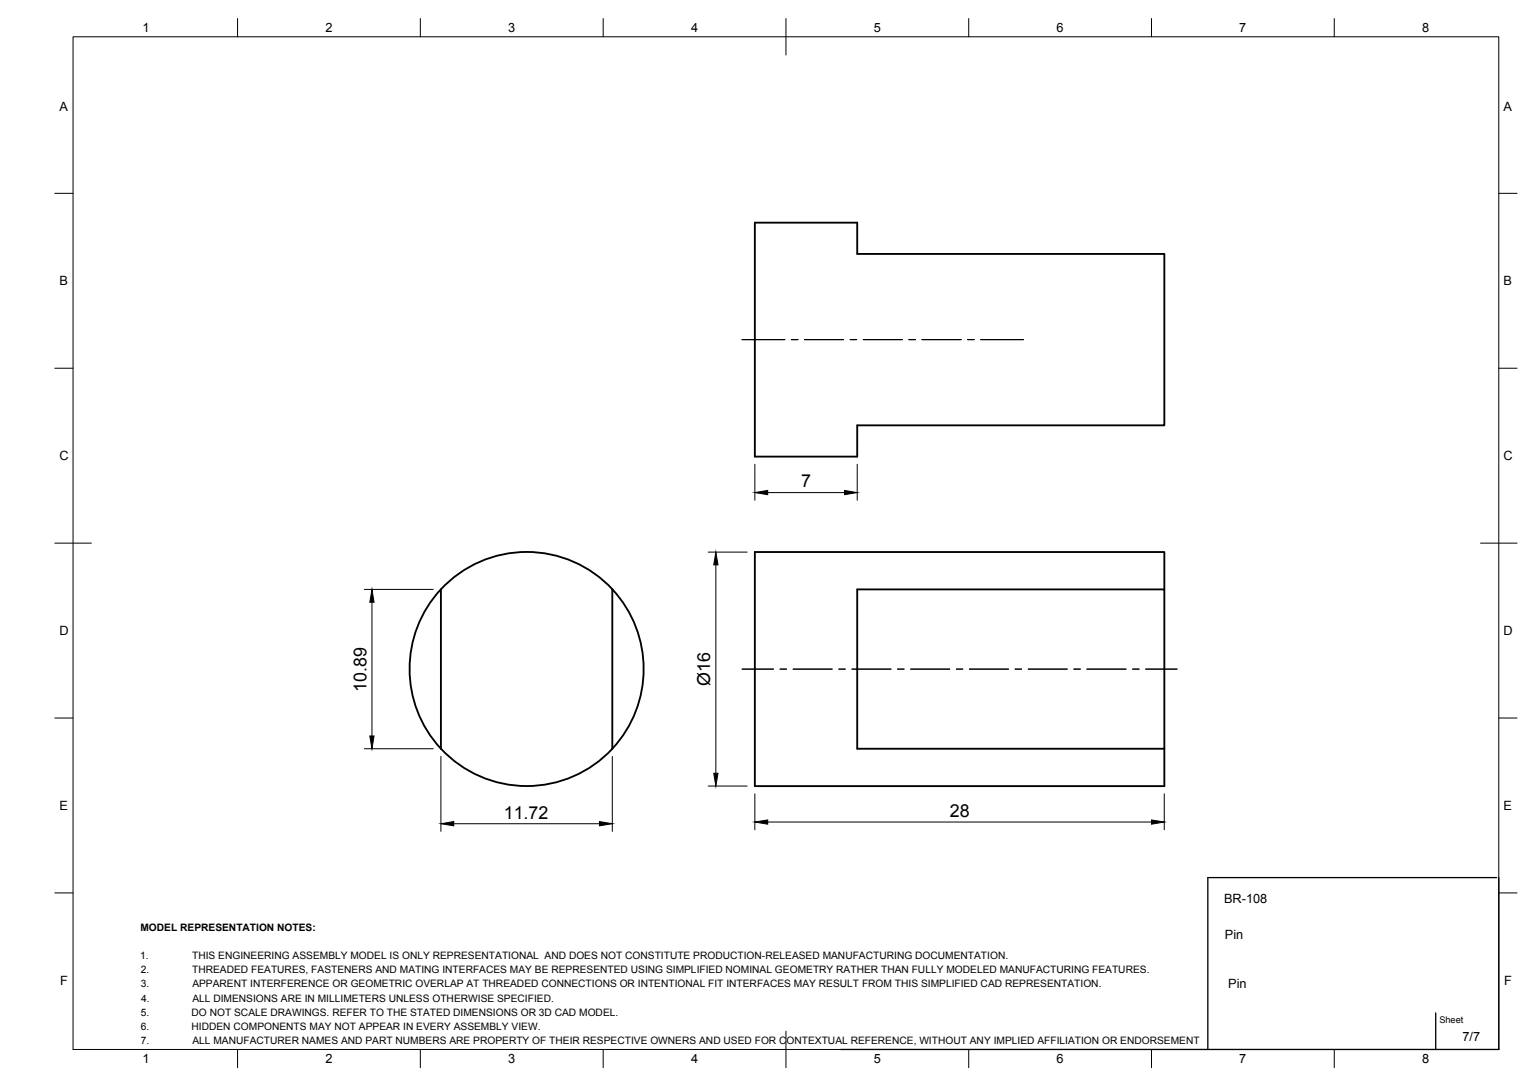
ISO-10303-21;
HEADER;
/* Generated by software containing ST-Developer
 * from STEP Tools, Inc. (www.steptools.com) 
 */

FILE_DESCRIPTION(
/* description */ (''),
/* implementation_level */ '2;1');

FILE_NAME(
/* name */ 'Pin.step',
/* time_stamp */ '2026-11-14T03:52:36-08:00',
/* author */ (''),
/* organization */ (''),
/* preprocessor_version */ 'ST-DEVELOPER v20.2',
/* originating_system */ 'Autodesk Translation Framework v15.17.0.0',
/* authorisation */ '');

FILE_SCHEMA (('AUTOMOTIVE_DESIGN { 1 0 10303 214 3 1 1 }'));
ENDSEC;

DATA;
#10=MECHANICAL_DESIGN_GEOMETRIC_PRESENTATION_REPRESENTATION('',(#197),#19443);
#181=SHAPE_REPRESENTATION_RELATIONSHIP('SRR','None',#19481,#189);
#189=ADVANCED_BREP_SHAPE_REPRESENTATION('',(#205),#19441);
#197=STYLED_ITEM('',(#19525),#205);
#205=MANIFOLD_SOLID_BREP('Body1',#2024);
#259=PLANE('',#2233);
#260=PLANE('',#2235);
#261=PLANE('',#2237);
#262=PLANE('',#2239);
#263=PLANE('',#2244);
#264=PLANE('',#2245);
#353=FACE_OUTER_BOUND('',#460,.T.);
#354=FACE_OUTER_BOUND('',#461,.T.);
#355=FACE_OUTER_BOUND('',#462,.T.);
#356=FACE_OUTER_BOUND('',#463,.T.);
#357=FACE_OUTER_BOUND('',#464,.T.);
#358=FACE_OUTER_BOUND('',#465,.T.);
#359=FACE_OUTER_BOUND('',#466,.T.);
#460=EDGE_LOOP('',(#1813,#1814));
#461=EDGE_LOOP('',(#1815,#1816));
#462=EDGE_LOOP('',(#1817));
#463=EDGE_LOOP('',(#1818,#1819,#1820,#1821));
#464=EDGE_LOOP('',(#1822,#1823,#1824,#1825,#1826,#1827,#1828,#1829,#1830,
#1831,#1832,#1833));
#465=EDGE_LOOP('',(#1834,#1835,#1836,#1837));
#466=EDGE_LOOP('',(#1838,#1839,#1840,#1841,#1842));
#577=LINE('',#19342,#704);
#578=LINE('',#19347,#705);
#579=LINE('',#19354,#706);
#580=LINE('',#19356,#707);
#581=LINE('',#19357,#708);
#582=LINE('',#19363,#709);
#583=LINE('',#19365,#710);
#584=LINE('',#19367,#711);
#585=LINE('',#19369,#712);
#704=VECTOR('',#2603,10.);
#705=VECTOR('',#2608,10.);
#706=VECTOR('',#2617,10.);
#707=VECTOR('',#2618,10.);
#708=VECTOR('',#2619,10.);
#709=VECTOR('',#2626,10.);
#710=VECTOR('',#2627,10.);
#711=VECTOR('',#2630,8.);
#712=VECTOR('',#2633,10.);
#768=CIRCLE('',#2234,8.);
#769=CIRCLE('',#2236,8.);
#770=CIRCLE('',#2238,8.);
#771=CIRCLE('',#2241,8.);
#772=CIRCLE('',#2242,8.);
#773=CIRCLE('',#2243,8.);
#970=VERTEX_POINT('',#19340);
#971=VERTEX_POINT('',#19341);
#972=VERTEX_POINT('',#19345);
#973=VERTEX_POINT('',#19346);
#974=VERTEX_POINT('',#19350);
#975=VERTEX_POINT('',#19353);
#976=VERTEX_POINT('',#19355);
#977=VERTEX_POINT('',#19359);
#978=VERTEX_POINT('',#19361);
#979=VERTEX_POINT('',#19364);
#1255=EDGE_CURVE('',#970,#971,#577,.T.);
#1256=EDGE_CURVE('',#971,#970,#768,.T.);
#1257=EDGE_CURVE('',#972,#973,#578,.T.);
#1258=EDGE_CURVE('',#973,#972,#769,.T.);
#1259=EDGE_CURVE('',#974,#974,#770,.T.);
#1260=EDGE_CURVE('',#970,#975,#579,.T.);
#1261=EDGE_CURVE('',#976,#975,#580,.T.);
#1262=EDGE_CURVE('',#971,#976,#581,.T.);
#1263=EDGE_CURVE('',#975,#977,#771,.T.);
#1264=EDGE_CURVE('',#978,#976,#772,.T.);
#1265=EDGE_CURVE('',#972,#978,#582,.T.);
#1266=EDGE_CURVE('',#973,#979,#583,.T.);
#1267=EDGE_CURVE('',#977,#979,#773,.T.);
#1268=EDGE_CURVE('',#977,#974,#584,.T.);
#1269=EDGE_CURVE('',#979,#978,#585,.T.);
#1813=ORIENTED_EDGE('',*,*,#1255,.T.);
#1814=ORIENTED_EDGE('',*,*,#1256,.T.);
#1815=ORIENTED_EDGE('',*,*,#1257,.T.);
#1816=ORIENTED_EDGE('',*,*,#1258,.T.);
#1817=ORIENTED_EDGE('',*,*,#1259,.T.);
#1818=ORIENTED_EDGE('',*,*,#1255,.F.);
#1819=ORIENTED_EDGE('',*,*,#1260,.T.);
#1820=ORIENTED_EDGE('',*,*,#1261,.F.);
#1821=ORIENTED_EDGE('',*,*,#1262,.F.);
#1822=ORIENTED_EDGE('',*,*,#1263,.F.);
#1823=ORIENTED_EDGE('',*,*,#1260,.F.);
#1824=ORIENTED_EDGE('',*,*,#1256,.F.);
#1825=ORIENTED_EDGE('',*,*,#1262,.T.);
#1826=ORIENTED_EDGE('',*,*,#1264,.F.);
#1827=ORIENTED_EDGE('',*,*,#1265,.F.);
#1828=ORIENTED_EDGE('',*,*,#1258,.F.);
#1829=ORIENTED_EDGE('',*,*,#1266,.T.);
#1830=ORIENTED_EDGE('',*,*,#1267,.F.);
#1831=ORIENTED_EDGE('',*,*,#1268,.T.);
#1832=ORIENTED_EDGE('',*,*,#1259,.F.);
#1833=ORIENTED_EDGE('',*,*,#1268,.F.);
#1834=ORIENTED_EDGE('',*,*,#1257,.F.);
#1835=ORIENTED_EDGE('',*,*,#1265,.T.);
#1836=ORIENTED_EDGE('',*,*,#1269,.F.);
#1837=ORIENTED_EDGE('',*,*,#1266,.F.);
#1838=ORIENTED_EDGE('',*,*,#1263,.T.);
#1839=ORIENTED_EDGE('',*,*,#1267,.T.);
#1840=ORIENTED_EDGE('',*,*,#1269,.T.);
#1841=ORIENTED_EDGE('',*,*,#1264,.T.);
#1842=ORIENTED_EDGE('',*,*,#1261,.T.);
#1920=CYLINDRICAL_SURFACE('',#2240,8.);
#2002=ADVANCED_FACE('',(#353),#259,.T.);
#2003=ADVANCED_FACE('',(#354),#260,.T.);
#2004=ADVANCED_FACE('',(#355),#261,.F.);
#2005=ADVANCED_FACE('',(#356),#262,.T.);
#2006=ADVANCED_FACE('',(#357),#1920,.T.);
#2007=ADVANCED_FACE('',(#358),#263,.T.);
#2008=ADVANCED_FACE('',(#359),#264,.T.);
#2024=CLOSED_SHELL('',(#2002,#2003,#2004,#2005,#2006,#2007,#2008));
#2232=AXIS2_PLACEMENT_3D('',#19338,#2599,#2600);
#2233=AXIS2_PLACEMENT_3D('',#19339,#2601,#2602);
#2234=AXIS2_PLACEMENT_3D('',#19343,#2604,#2605);
#2235=AXIS2_PLACEMENT_3D('',#19344,#2606,#2607);
#2236=AXIS2_PLACEMENT_3D('',#19348,#2609,#2610);
#2237=AXIS2_PLACEMENT_3D('',#19349,#2611,#2612);
#2238=AXIS2_PLACEMENT_3D('',#19351,#2613,#2614);
#2239=AXIS2_PLACEMENT_3D('',#19352,#2615,#2616);
#2240=AXIS2_PLACEMENT_3D('',#19358,#2620,#2621);
#2241=AXIS2_PLACEMENT_3D('',#19360,#2622,#2623);
#2242=AXIS2_PLACEMENT_3D('',#19362,#2624,#2625);
#2243=AXIS2_PLACEMENT_3D('',#19366,#2628,#2629);
#2244=AXIS2_PLACEMENT_3D('',#19368,#2631,#2632);
#2245=AXIS2_PLACEMENT_3D('',#19370,#2634,#2635);
#2599=DIRECTION('axis',(0.,0.,1.));
#2600=DIRECTION('refdir',(1.,0.,0.));
#2601=DIRECTION('center_axis',(0.,0.,-1.));
#2602=DIRECTION('ref_axis',(1.,0.,0.));
#2603=DIRECTION('',(1.,0.,0.));
#2604=DIRECTION('center_axis',(0.,0.,-1.));
#2605=DIRECTION('ref_axis',(1.,0.,0.));
#2606=DIRECTION('center_axis',(0.,0.,-1.));
#2607=DIRECTION('ref_axis',(1.,0.,0.));
#2608=DIRECTION('',(-1.,0.,0.));
#2609=DIRECTION('center_axis',(0.,0.,-1.));
#2610=DIRECTION('ref_axis',(1.,0.,0.));
#2611=DIRECTION('center_axis',(0.,0.,-1.));
#2612=DIRECTION('ref_axis',(1.,0.,0.));
#2613=DIRECTION('center_axis',(0.,0.,1.));
#2614=DIRECTION('ref_axis',(1.,0.,0.));
#2615=DIRECTION('center_axis',(0.,-1.,0.));
#2616=DIRECTION('ref_axis',(-1.,0.,0.));
#2617=DIRECTION('',(0.,0.,-1.));
#2618=DIRECTION('',(-1.,0.,0.));
#2619=DIRECTION('',(0.,0.,-1.));
#2620=DIRECTION('center_axis',(0.,0.,-1.));
#2621=DIRECTION('ref_axis',(1.,0.,0.));
#2622=DIRECTION('center_axis',(0.,0.,-1.));
#2623=DIRECTION('ref_axis',(1.,0.,0.));
#2624=DIRECTION('center_axis',(0.,0.,-1.));
#2625=DIRECTION('ref_axis',(1.,0.,0.));
#2626=DIRECTION('',(0.,0.,-1.));
#2627=DIRECTION('',(0.,0.,-1.));
#2628=DIRECTION('center_axis',(0.,0.,-1.));
#2629=DIRECTION('ref_axis',(1.,0.,0.));
#2630=DIRECTION('',(0.,0.,1.));
#2631=DIRECTION('center_axis',(0.,1.,0.));
#2632=DIRECTION('ref_axis',(1.,0.,0.));
#2633=DIRECTION('',(1.,0.,0.));
#2634=DIRECTION('center_axis',(0.,0.,-1.));
#2635=DIRECTION('ref_axis',(1.,0.,0.));
#19338=CARTESIAN_POINT('',(0.,0.,0.));
#19339=CARTESIAN_POINT('Origin',(0.,0.,0.));
#19340=CARTESIAN_POINT('',(-5.44687084534895,-5.85931719521034,0.));
#19341=CARTESIAN_POINT('',(5.44687084534894,-5.85931719521034,0.));
#19342=CARTESIAN_POINT('',(-17.7281904880723,-5.85931719521034,0.));
#19343=CARTESIAN_POINT('Origin',(0.,0.,0.));
#19344=CARTESIAN_POINT('Origin',(0.,0.,0.));
#19345=CARTESIAN_POINT('',(5.44687084534895,5.85931719521034,0.));
#19346=CARTESIAN_POINT('',(-5.44687084534894,5.85931719521034,0.));
#19347=CARTESIAN_POINT('',(17.7281904880723,5.85931719521034,0.));
#19348=CARTESIAN_POINT('Origin',(0.,0.,0.));
#19349=CARTESIAN_POINT('Origin',(0.,0.,7.));
#19350=CARTESIAN_POINT('',(-8.,9.79717439317882E-16,7.));
#19351=CARTESIAN_POINT('Origin',(0.,0.,7.));
#19352=CARTESIAN_POINT('Origin',(5.44687084534894,-5.85931719521034,0.));
#19353=CARTESIAN_POINT('',(-5.44687084534895,-5.85931719521034,-21.));
#19354=CARTESIAN_POINT('',(-5.44687084534895,-5.85931719521034,0.));
#19355=CARTESIAN_POINT('',(5.44687084534894,-5.85931719521034,-21.));
#19356=CARTESIAN_POINT('',(-17.7281904880723,-5.85931719521034,-21.));
#19357=CARTESIAN_POINT('',(5.44687084534894,-5.85931719521034,0.));
#19358=CARTESIAN_POINT('Origin',(0.,0.,0.));
#19359=CARTESIAN_POINT('',(-8.,9.79717439317883E-16,-21.));
#19360=CARTESIAN_POINT('Origin',(0.,0.,-21.));
#19361=CARTESIAN_POINT('',(5.44687084534895,5.85931719521034,-21.));
#19362=CARTESIAN_POINT('Origin',(0.,0.,-21.));
#19363=CARTESIAN_POINT('',(5.44687084534895,5.85931719521034,0.));
#19364=CARTESIAN_POINT('',(-5.44687084534894,5.85931719521034,-21.));
#19365=CARTESIAN_POINT('',(-5.44687084534894,5.85931719521034,0.));
#19366=CARTESIAN_POINT('Origin',(0.,0.,-21.));
#19367=CARTESIAN_POINT('',(-8.,9.79717439317883E-16,0.));
#19368=CARTESIAN_POINT('Origin',(-5.44687084534894,5.85931719521034,0.));
#19369=CARTESIAN_POINT('',(17.7281904880723,5.85931719521034,-21.));
#19370=CARTESIAN_POINT('Origin',(0.,0.,-21.));
#19431=UNCERTAINTY_MEASURE_WITH_UNIT(LENGTH_MEASURE(0.01),#19444,
'DISTANCE_ACCURACY_VALUE',
'Maximum model space distance between geometric entities at asserted c
onnectivities');
#19433=UNCERTAINTY_MEASURE_WITH_UNIT(LENGTH_MEASURE(0.01),#19444,
'DISTANCE_ACCURACY_VALUE',
'Maximum model space distance between geometric entities at asserted c
onnectivities');
#19441=(
GEOMETRIC_REPRESENTATION_CONTEXT(3)
GLOBAL_UNCERTAINTY_ASSIGNED_CONTEXT((#19431))
GLOBAL_UNIT_ASSIGNED_CONTEXT((#19444,#19446,#19447))
REPRESENTATION_CONTEXT('','3D')
);
#19443=(
GEOMETRIC_REPRESENTATION_CONTEXT(3)
GLOBAL_UNCERTAINTY_ASSIGNED_CONTEXT((#19433))
GLOBAL_UNIT_ASSIGNED_CONTEXT((#19444,#19446,#19447))
REPRESENTATION_CONTEXT('','3D')
);
#19444=(
LENGTH_UNIT()
NAMED_UNIT(*)
SI_UNIT(.MILLI.,.METRE.)
);
#19446=(
NAMED_UNIT(*)
PLANE_ANGLE_UNIT()
SI_UNIT($,.RADIAN.)
);
#19447=(
NAMED_UNIT(*)
SI_UNIT($,.STERADIAN.)
SOLID_ANGLE_UNIT()
);
#19455=SHAPE_DEFINITION_REPRESENTATION(#19464,#19481);
#19464=PRODUCT_DEFINITION_SHAPE('',$,#19491);
#19481=SHAPE_REPRESENTATION('',(#2232),#19441);
#19483=PRODUCT_DEFINITION_CONTEXT('part definition',#19512,'design');
#19491=PRODUCT_DEFINITION('Pin','Pin',#19500,#19483);
#19500=PRODUCT_DEFINITION_FORMATION('',$,#19521);
#19512=APPLICATION_CONTEXT(
'Core Data for Automotive Mechanical Design Process');
#19513=PRODUCT_CONTEXT('part definition',#19512,'mechanical');
#19521=PRODUCT('Pin','Pin',$,(#19513));
#19525=PRESENTATION_STYLE_ASSIGNMENT((#19528));
#19528=SURFACE_STYLE_USAGE(.BOTH.,#19531);
#19531=SURFACE_SIDE_STYLE('',(#19534));
#19534=SURFACE_STYLE_FILL_AREA(#19537);
#19537=FILL_AREA_STYLE('Opaque(160,160,160)',(#19540));
#19540=FILL_AREA_STYLE_COLOUR('Opaque(160,160,160)',#19543);
#19543=COLOUR_RGB('Opaque(160,160,160)',0.627450980392157,0.627450980392157,
0.627450980392157);
ENDSEC;
END-ISO-10303-21;
